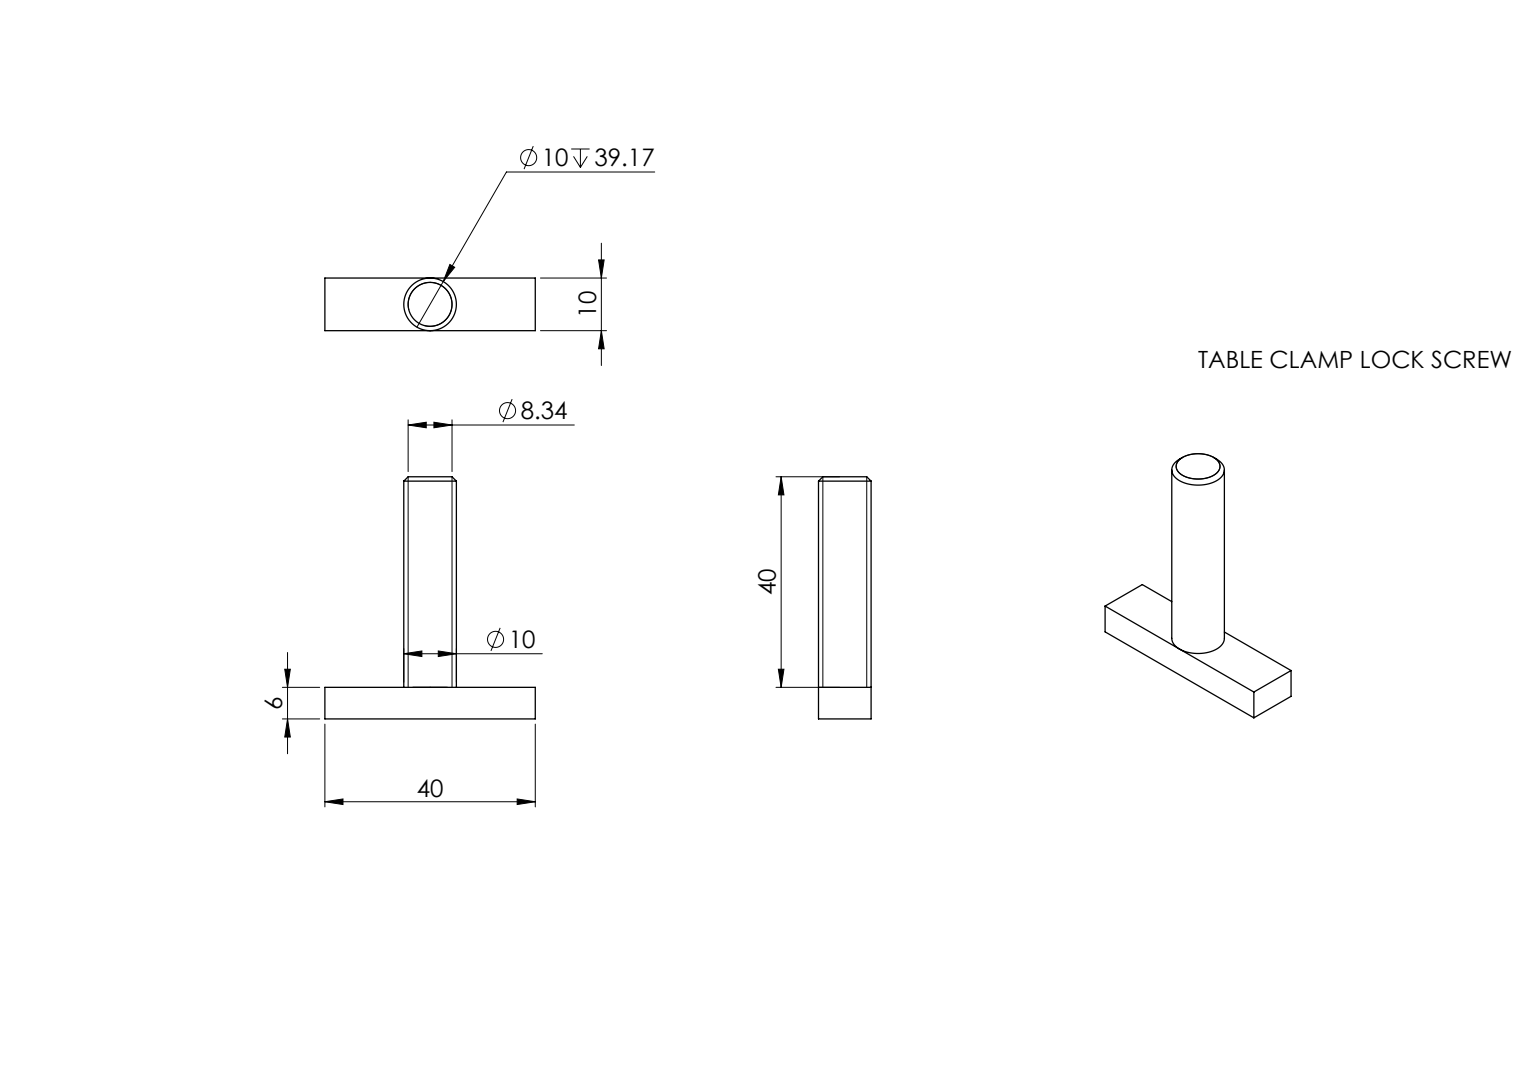
ISO-10303-21;
HEADER;
FILE_DESCRIPTION (('STEP AP214'),
    '1' );
FILE_NAME ('Table Clamp Lock Screw.step',
    '2026-10-22T10:02:39',
    ( '' ),
    ( '' ),
    'SwSTEP 2.0',
    'SolidWorks 2026',
    '' );
FILE_SCHEMA (( 'AUTOMOTIVE_DESIGN' ));
ENDSEC;

DATA;
#63=ADVANCED_FACE ( 'NONE', ( #6296 ), #11663, .F. ) ;
#65=DIRECTION ( 'NONE',  ( -0.000000000000000000, -1.000000000000000000, -0.000000000000000000 ) ) ;
#81=COLOUR_RGB ( '',0.8941176470588234615, 0.8941176470588234615, 0.8941176470588234615 ) ;
#86=LINE ( 'NONE', #1108, #4140 ) ;
#156=DIRECTION ( 'NONE',  ( -0.000000000000000000, -1.000000000000000000, -0.000000000000000000 ) ) ;
#174=FACE_OUTER_BOUND ( 'NONE', #11292, .T. ) ;
#257=( NAMED_UNIT ( * ) SI_UNIT ( $, .STERADIAN. ) SOLID_ANGLE_UNIT ( ) );
#287=DIRECTION ( 'NONE',  ( 0.000000000000000000, 0.000000000000000000, -1.000000000000000000 ) ) ;
#300=CARTESIAN_POINT ( 'NONE',  ( -20.00000000000003197, -57.00000000000000000, 5.000000000000000000 ) ) ;
#357=FACE_OUTER_BOUND ( 'NONE', #4501, .T. ) ;
#394=UNCERTAINTY_MEASURE_WITH_UNIT (LENGTH_MEASURE( 1.000000000000000082E-05 ), #5013, 'distance_accuracy_value', 'NONE');
#416=CLOSED_SHELL ( 'NONE', ( #7269, #9582, #2198, #63, #11043, #9304, #2244, #10765, #4629, #4313, #3244, #8345 ) ) ;
#432=EDGE_CURVE ( 'NONE', #3322, #5122, #11360, .T. ) ;
#533=CARTESIAN_POINT ( 'NONE',  ( -20.00000000000003197, -63.00000000000000000, 5.000000000000000000 ) ) ;
#646=DIRECTION ( 'NONE',  ( 0.000000000000000000, 0.000000000000000000, 1.000000000000000000 ) ) ;
#657=CARTESIAN_POINT ( 'NONE',  ( 0.000000000000000000, -57.00000000000000000, 0.000000000000000000 ) ) ;
#733=EDGE_CURVE ( 'NONE', #9917, #5658, #853, .T. ) ;
#777=DIRECTION ( 'NONE',  ( -0.000000000000000000, -1.000000000000000000, -0.000000000000000000 ) ) ;
#844=( GEOMETRIC_REPRESENTATION_CONTEXT ( 3 ) GLOBAL_UNCERTAINTY_ASSIGNED_CONTEXT ( ( #5921 ) ) GLOBAL_UNIT_ASSIGNED_CONTEXT ( ( #5850, #10497, #257 ) ) REPRESENTATION_CONTEXT ( 'NONE', 'WORKASPACE' ) );
#853=CIRCLE ( 'NONE', #2783, 4.171999999999999709 ) ;
#865=FACE_OUTER_BOUND ( 'NONE', #7245, .T. ) ;
#905=LINE ( 'NONE', #4465, #8956 ) ;
#995=ORIENTED_EDGE ( 'NONE', *, *, #8595, .F. ) ;
#1001=CARTESIAN_POINT ( 'NONE',  ( 0.000000000000000000, -17.82799999999998875, 0.000000000000000000 ) ) ;
#1089=CARTESIAN_POINT ( 'NONE',  ( 0.000000000000000000, -17.82799999999998875, -4.999999999999995559 ) ) ;
#1094=ORIENTED_EDGE ( 'NONE', *, *, #432, .T. ) ;
#1108=CARTESIAN_POINT ( 'NONE',  ( -20.00000000000003197, -57.00000000000000000, 5.000000000000000000 ) ) ;
#1155=AXIS2_PLACEMENT_3D ( 'NONE', #5306, #2664, #4410 ) ;
#1159=VECTOR ( 'NONE', #10817, 1000.000000000000000 ) ;
#1182=EDGE_CURVE ( 'NONE', #3322, #7121, #8405, .T. ) ;
#1184=( NAMED_UNIT ( * ) SI_UNIT ( $, .STERADIAN. ) SOLID_ANGLE_UNIT ( ) );
#1255=FACE_OUTER_BOUND ( 'NONE', #2174, .T. ) ;
#1282=LINE ( 'NONE', #10265, #7592 ) ;
#1303=ORIENTED_EDGE ( 'NONE', *, *, #1182, .F. ) ;
#1305=CARTESIAN_POINT ( 'NONE',  ( 19.99999999999996803, -63.00000000000000000, 5.000000000000000000 ) ) ;
#1346=CARTESIAN_POINT ( 'NONE',  ( 0.000000000000000000, -17.82799999999998875, -4.999999999999995559 ) ) ;
#1347=SURFACE_STYLE_USAGE ( .BOTH. , #2122 ) ;
#1383=DIRECTION ( 'NONE',  ( 1.000000000000000000, 0.000000000000000000, 0.000000000000000000 ) ) ;
#1405=FILL_AREA_STYLE ('',( #5909 ) ) ;
#1440=STYLED_ITEM ( 'NONE', ( #5732 ), #4566 ) ;
#1453=PRODUCT ( 'Table Clamp Lock Screw', 'Table Clamp Lock Screw', '', ( #9179 ) ) ;
#1565=ORIENTED_EDGE ( 'NONE', *, *, #10552, .T. ) ;
#1669=ORIENTED_EDGE ( 'NONE', *, *, #5875, .F. ) ;
#1676=CYLINDRICAL_SURFACE ( 'NONE', #10532, 4.999999999999997335 ) ;
#1688=ORIENTED_EDGE ( 'NONE', *, *, #5113, .T. ) ;
#1701=CARTESIAN_POINT ( 'NONE',  ( -20.00000000000003197, -63.00000000000000000, 5.000000000000000000 ) ) ;
#1708=CARTESIAN_POINT ( 'NONE',  ( 0.000000000000000000, -17.82799999999998875, 0.000000000000000000 ) ) ;
#1723=DIRECTION ( 'NONE',  ( -0.000000000000000000, -0.000000000000000000, -1.000000000000000000 ) ) ;
#1787=PLANE ( 'NONE',  #11606 ) ;
#1877=MECHANICAL_DESIGN_GEOMETRIC_PRESENTATION_REPRESENTATION('',(#6123),#11251);
#1892=ORIENTED_EDGE ( 'NONE', *, *, #4690, .T. ) ;
#1924=CARTESIAN_POINT ( 'NONE',  ( 6.123233995736761352E-16, -17.82799999999998875, 4.999999999999995559 ) ) ;
#2039=VECTOR ( 'NONE', #4198, 1000.000000000000000 ) ;
#2087=CARTESIAN_POINT ( 'NONE',  ( 0.000000000000000000, -17.82799999999998875, 0.000000000000000000 ) ) ;
#2122=SURFACE_SIDE_STYLE ('',( #9552 ) ) ;
#2174=EDGE_LOOP ( 'NONE', ( #11721, #10327, #3071, #9481 ) ) ;
#2197=PRODUCT_DEFINITION ( 'UNKNOWN', '', #10978, #3306 ) ;
#2198=ADVANCED_FACE ( 'NONE', ( #9905 ), #2546, .F. ) ;
#2216=EDGE_CURVE ( 'NONE', #2768, #9929, #10794, .T. ) ;
#2225=CIRCLE ( 'NONE', #4337, 4.171999999999999709 ) ;
#2244=ADVANCED_FACE ( 'NONE', ( #2605 ), #2729, .F. ) ;
#2410=ORIENTED_EDGE ( 'NONE', *, *, #8591, .F. ) ;
#2460=DIRECTION ( 'NONE',  ( -0.000000000000000000, -1.000000000000000000, -0.000000000000000000 ) ) ;
#2467=VECTOR ( 'NONE', #4475, 1000.000000000000000 ) ;
#2546=PLANE ( 'NONE',  #1155 ) ;
#2603=VERTEX_POINT ( 'NONE', #8563 ) ;
#2605=FACE_OUTER_BOUND ( 'NONE', #8879, .T. ) ;
#2664=DIRECTION ( 'NONE',  ( 0.000000000000000000, -1.000000000000000000, 0.000000000000000000 ) ) ;
#2671=EDGE_LOOP ( 'NONE', ( #8662, #1669, #10822, #1688 ) ) ;
#2696=ORIENTED_EDGE ( 'NONE', *, *, #11695, .T. ) ;
#2705=AXIS2_PLACEMENT_3D ( 'NONE', #6076, #10774, #8759 ) ;
#2729=PLANE ( 'NONE',  #7869 ) ;
#2768=VERTEX_POINT ( 'NONE', #1305 ) ;
#2783=AXIS2_PLACEMENT_3D ( 'NONE', #5496, #9145, #3695 ) ;
#2840=ORIENTED_EDGE ( 'NONE', *, *, #5067, .T. ) ;
#2859=CARTESIAN_POINT ( 'NONE',  ( 6.123233995736761352E-16, -17.82799999999998875, 4.999999999999995559 ) ) ;
#2946=EDGE_CURVE ( 'NONE', #9538, #5122, #7903, .T. ) ;
#2953=VECTOR ( 'NONE', #10579, 1000.000000000000000 ) ;
#3042=DIRECTION ( 'NONE',  ( -0.000000000000000000, -0.000000000000000000, -1.000000000000000000 ) ) ;
#3062=EDGE_CURVE ( 'NONE', #5122, #6726, #11232, .T. ) ;
#3071=ORIENTED_EDGE ( 'NONE', *, *, #9421, .F. ) ;
#3083=EDGE_CURVE ( 'NONE', #3150, #2603, #5811, .T. ) ;
#3089=( NAMED_UNIT ( * ) SI_UNIT ( $, .STERADIAN. ) SOLID_ANGLE_UNIT ( ) );
#3101=CARTESIAN_POINT ( 'NONE',  ( 19.99999999999996803, -57.00000000000000000, 5.000000000000000000 ) ) ;
#3108=( LENGTH_UNIT ( ) NAMED_UNIT ( * ) SI_UNIT ( .MILLI., .METRE. ) );
#3150=VERTEX_POINT ( 'NONE', #10342 ) ;
#3180=DIRECTION ( 'NONE',  ( -1.000000000000000000, 0.000000000000000000, -0.000000000000000000 ) ) ;
#3207=VERTEX_POINT ( 'NONE', #5199 ) ;
#3232=ORIENTED_EDGE ( 'NONE', *, *, #5875, .T. ) ;
#3244=ADVANCED_FACE ( 'NONE', ( #10687 ), #3557, .T. ) ;
#3264=VECTOR ( 'NONE', #3560, 1000.000000000000000 ) ;
#3306=PRODUCT_DEFINITION_CONTEXT ( 'detailed design', #10813, 'design' ) ;
#3322=VERTEX_POINT ( 'NONE', #1346 ) ;
#3442=CARTESIAN_POINT ( 'NONE',  ( 19.99999999999996803, -63.00000000000000000, 5.000000000000000000 ) ) ;
#3482=FACE_OUTER_BOUND ( 'NONE', #11135, .T. ) ;
#3511=LINE ( 'NONE', #7126, #2467 ) ;
#3544=( GEOMETRIC_REPRESENTATION_CONTEXT ( 3 ) GLOBAL_UNCERTAINTY_ASSIGNED_CONTEXT ( ( #394 ) ) GLOBAL_UNIT_ASSIGNED_CONTEXT ( ( #5013, #7644, #3089 ) ) REPRESENTATION_CONTEXT ( 'NONE', 'WORKASPACE' ) );
#3557=CONICAL_SURFACE ( 'NONE', #10242, 4.999999999999995559, 0.7853981633974530530 ) ;
#3560=DIRECTION ( 'NONE',  ( 0.000000000000000000, 1.000000000000000000, 0.000000000000000000 ) ) ;
#3591=EDGE_CURVE ( 'NONE', #9484, #9538, #1282, .T. ) ;
#3667=AXIS2_PLACEMENT_3D ( 'NONE', #5628, #156, #9508 ) ;
#3695=DIRECTION ( 'NONE',  ( 0.000000000000000000, 0.000000000000000000, -1.000000000000000000 ) ) ;
#3708=DIRECTION ( 'NONE',  ( 0.000000000000000000, -1.000000000000000000, 0.000000000000000000 ) ) ;
#3713=ORIENTED_EDGE ( 'NONE', *, *, #8804, .F. ) ;
#3749=DIRECTION ( 'NONE',  ( -1.000000000000000000, -0.000000000000000000, -0.000000000000000000 ) ) ;
#3761=CONICAL_SURFACE ( 'NONE', #5303, 4.999999999999995559, 0.7853981633974530530 ) ;
#3772=VECTOR ( 'NONE', #6533, 1000.000000000000000 ) ;
#3807=EDGE_CURVE ( 'NONE', #7121, #3322, #8159, .T. ) ;
#3818=ORIENTED_EDGE ( 'NONE', *, *, #3807, .T. ) ;
#3842=PLANE ( 'NONE',  #10150 ) ;
#3896=ORIENTED_EDGE ( 'NONE', *, *, #2216, .T. ) ;
#4021=CARTESIAN_POINT ( 'NONE',  ( 4.171999999999999709, -17.00000000000000000, 0.000000000000000000 ) ) ;
#4023=PLANE ( 'NONE',  #6481 ) ;
#4081=CARTESIAN_POINT ( 'NONE',  ( 0.000000000000000000, 0.000000000000000000, 5.000000000000000000 ) ) ;
#4122=CARTESIAN_POINT ( 'NONE',  ( 0.000000000000000000, -57.00000000000000000, -4.999999999999997335 ) ) ;
#4140=VECTOR ( 'NONE', #3749, 1000.000000000000000 ) ;
#4148=AXIS2_PLACEMENT_3D ( 'NONE', #7916, #5830, #6905 ) ;
#4172=SHAPE_REPRESENTATION ( 'Table Clamp Lock Screw', ( #4738 ), #844 ) ;
#4198=DIRECTION ( 'NONE',  ( -0.000000000000000000, -1.000000000000000000, -0.000000000000000000 ) ) ;
#4205=DIRECTION ( 'NONE',  ( 0.000000000000000000, 0.000000000000000000, -1.000000000000000000 ) ) ;
#4206=ORIENTED_EDGE ( 'NONE', *, *, #7278, .F. ) ;
#4265=DIRECTION ( 'NONE',  ( -0.000000000000000000, -1.000000000000000000, -0.000000000000000000 ) ) ;
#4281=DIRECTION ( 'NONE',  ( 0.000000000000000000, 0.000000000000000000, -1.000000000000000000 ) ) ;
#4295=CARTESIAN_POINT ( 'NONE',  ( 19.99999999999996803, -57.00000000000000000, 5.000000000000000000 ) ) ;
#4313=ADVANCED_FACE ( 'NONE', ( #174 ), #3842, .T. ) ;
#4337=AXIS2_PLACEMENT_3D ( 'NONE', #11160, #65, #8471 ) ;
#4357=ORIENTED_EDGE ( 'NONE', *, *, #3062, .T. ) ;
#4374=VECTOR ( 'NONE', #7623, 1000.000000000000000 ) ;
#4410=DIRECTION ( 'NONE',  ( 0.000000000000000000, -0.000000000000000000, -1.000000000000000000 ) ) ;
#4416=DIRECTION ( 'NONE',  ( -0.000000000000000000, -1.000000000000000000, -0.000000000000000000 ) ) ;
#4465=CARTESIAN_POINT ( 'NONE',  ( -20.00000000000003197, -63.00000000000000000, 5.000000000000000000 ) ) ;
#4475=DIRECTION ( 'NONE',  ( -0.000000000000000000, -0.000000000000000000, -1.000000000000000000 ) ) ;
#4501=EDGE_LOOP ( 'NONE', ( #3896, #5187, #1565, #9674, #2696 ) ) ;
#4518=ORIENTED_EDGE ( 'NONE', *, *, #8804, .T. ) ;
#4566=ADVANCED_BREP_SHAPE_REPRESENTATION ( '', ( #4740, #4738 ), #844 ) ;
#4603=DIRECTION ( 'NONE',  ( 0.000000000000000000, 0.000000000000000000, -1.000000000000000000 ) ) ;
#4629=ADVANCED_FACE ( 'NONE', ( #10941 ), #7142, .T. ) ;
#4636=ORIENTED_EDGE ( 'NONE', *, *, #9664, .F. ) ;
#4660=DIRECTION ( 'NONE',  ( 0.000000000000000000, 0.000000000000000000, -1.000000000000000000 ) ) ;
#4686=SHAPE_DEFINITION_REPRESENTATION ( #8071, #4172 ) ;
#4690=EDGE_CURVE ( 'NONE', #8651, #5122, #5392, .T. ) ;
#4724=CARTESIAN_POINT ( 'NONE',  ( 6.123233995736763324E-16, -57.00000000000000000, 4.999999999999997335 ) ) ;
#4738=AXIS2_PLACEMENT_3D ( 'NONE', #6164, #8011, #1383 ) ;
#4740=MANIFOLD_SOLID_BREP ( 'M10 Machine Threads Stud1', #416 ) ;
#4895=LINE ( 'NONE', #3101, #8810 ) ;
#5013=( LENGTH_UNIT ( ) NAMED_UNIT ( * ) SI_UNIT ( .MILLI., .METRE. ) );
#5020=AXIS2_PLACEMENT_3D ( 'NONE', #9927, #11725, #646 ) ;
#5067=EDGE_CURVE ( 'NONE', #2603, #9484, #11764, .T. ) ;
#5113=EDGE_CURVE ( 'NONE', #2768, #9484, #3511, .T. ) ;
#5122=VERTEX_POINT ( 'NONE', #9138 ) ;
#5187=ORIENTED_EDGE ( 'NONE', *, *, #8591, .T. ) ;
#5199=CARTESIAN_POINT ( 'NONE',  ( -20.00000000000003197, -57.00000000000000000, 5.000000000000000000 ) ) ;
#5236=CARTESIAN_POINT ( 'NONE',  ( -20.00000000000003197, -63.00000000000000000, -5.000000000000000000 ) ) ;
#5257=DIRECTION ( 'NONE',  ( 0.000000000000000000, 0.000000000000000000, -1.000000000000000000 ) ) ;
#5303=AXIS2_PLACEMENT_3D ( 'NONE', #1001, #10099, #4660 ) ;
#5306=CARTESIAN_POINT ( 'NONE',  ( -20.00000000000003197, -57.00000000000000000, 5.000000000000000000 ) ) ;
#5317=CARTESIAN_POINT ( 'NONE',  ( -20.00000000000003197, -63.00000000000000000, -5.000000000000000000 ) ) ;
#5362=CARTESIAN_POINT ( 'NONE',  ( 0.000000000000000000, -17.82799999999998875, 0.000000000000000000 ) ) ;
#5392=CIRCLE ( 'NONE', #3667, 5.000000000000000000 ) ;
#5398=CARTESIAN_POINT ( 'NONE',  ( -20.00000000000003197, -57.00000000000000000, 5.000000000000000000 ) ) ;
#5496=CARTESIAN_POINT ( 'NONE',  ( 0.000000000000000000, -17.00000000000000000, 0.000000000000000000 ) ) ;
#5502=LINE ( 'NONE', #2859, #1159 ) ;
#5533=AXIS2_PLACEMENT_3D ( 'NONE', #2087, #8507, #287 ) ;
#5567=FACE_OUTER_BOUND ( 'NONE', #9764, .T. ) ;
#5628=CARTESIAN_POINT ( 'NONE',  ( 0.000000000000000000, -57.00000000000000000, 0.000000000000000000 ) ) ;
#5629=CARTESIAN_POINT ( 'NONE',  ( 19.99999999999996803, -57.00000000000000000, -5.000000000000000000 ) ) ;
#5633=UNCERTAINTY_MEASURE_WITH_UNIT (LENGTH_MEASURE( 1.000000000000000082E-05 ), #3108, 'distance_accuracy_value', 'NONE');
#5658=VERTEX_POINT ( 'NONE', #11600 ) ;
#5663=ORIENTED_EDGE ( 'NONE', *, *, #10552, .F. ) ;
#5691=LINE ( 'NONE', #4724, #3772 ) ;
#5732=PRESENTATION_STYLE_ASSIGNMENT (( #1347 ) ) ;
#5811=LINE ( 'NONE', #8619, #10807 ) ;
#5830=DIRECTION ( 'NONE',  ( 1.000000000000000000, 0.000000000000000000, 0.000000000000000000 ) ) ;
#5850=( LENGTH_UNIT ( ) NAMED_UNIT ( * ) SI_UNIT ( .MILLI., .METRE. ) );
#5875=EDGE_CURVE ( 'NONE', #9929, #9538, #4895, .T. ) ;
#5909=FILL_AREA_STYLE_COLOUR ( '', #81 ) ;
#5921=UNCERTAINTY_MEASURE_WITH_UNIT (LENGTH_MEASURE( 1.000000000000000082E-05 ), #5850, 'distance_accuracy_value', 'NONE');
#5926=CARTESIAN_POINT ( 'NONE',  ( -20.00000000000003197, -57.00000000000000000, -5.000000000000000000 ) ) ;
#5934=DIRECTION ( 'NONE',  ( -1.000000000000000000, -0.000000000000000000, -0.000000000000000000 ) ) ;
#6076=CARTESIAN_POINT ( 'NONE',  ( 0.000000000000000000, -57.00000000000000000, 0.000000000000000000 ) ) ;
#6084=ORIENTED_EDGE ( 'NONE', *, *, #11695, .F. ) ;
#6098=DIRECTION ( 'NONE',  ( -0.000000000000000000, -0.000000000000000000, -1.000000000000000000 ) ) ;
#6108=ORIENTED_EDGE ( 'NONE', *, *, #1182, .T. ) ;
#6123=STYLED_ITEM('',(#11895),#4740);
#6127=DIRECTION ( 'NONE',  ( 0.000000000000000000, 0.000000000000000000, -1.000000000000000000 ) ) ;
#6133=ORIENTED_EDGE ( 'NONE', *, *, #9063, .F. ) ;
#6164=CARTESIAN_POINT ( 'NONE',  ( 0.000000000000000000, 0.000000000000000000, 0.000000000000000000 ) ) ;
#6296=FACE_OUTER_BOUND ( 'NONE', #2671, .T. ) ;
#6358=AXIS2_PLACEMENT_3D ( 'NONE', #8874, #2460, #6127 ) ;
#6371=ORIENTED_EDGE ( 'NONE', *, *, #2946, .T. ) ;
#6386=DIRECTION ( 'NONE',  ( 0.000000000000000000, 1.000000000000000000, 0.000000000000000000 ) ) ;
#6409=DIRECTION ( 'NONE',  ( -1.000000000000000000, 0.000000000000000000, -0.000000000000000000 ) ) ;
#6481=AXIS2_PLACEMENT_3D ( 'NONE', #4081, #11371, #3180 ) ;
#6532=VECTOR ( 'NONE', #1723, 1000.000000000000000 ) ;
#6533=DIRECTION ( 'NONE',  ( -0.000000000000000000, -1.000000000000000000, -0.000000000000000000 ) ) ;
#6544=ORIENTED_EDGE ( 'NONE', *, *, #432, .F. ) ;
#6570=ORIENTED_EDGE ( 'NONE', *, *, #3591, .F. ) ;
#6626=DIRECTION ( 'NONE',  ( 0.000000000000000000, -0.000000000000000000, 1.000000000000000000 ) ) ;
#6726=VERTEX_POINT ( 'NONE', #11747 ) ;
#6732=DIRECTION ( 'NONE',  ( 0.000000000000000000, 1.000000000000000000, 0.000000000000000000 ) ) ;
#6763=ORIENTED_EDGE ( 'NONE', *, *, #3083, .T. ) ;
#6905=DIRECTION ( 'NONE',  ( 0.000000000000000000, 0.000000000000000000, -1.000000000000000000 ) ) ;
#7121=VERTEX_POINT ( 'NONE', #1924 ) ;
#7126=CARTESIAN_POINT ( 'NONE',  ( 19.99999999999996803, -63.00000000000000000, 5.000000000000000000 ) ) ;
#7129=ORIENTED_EDGE ( 'NONE', *, *, #733, .F. ) ;
#7142=PLANE ( 'NONE',  #8258 ) ;
#7205=DIRECTION ( 'NONE',  ( 0.000000000000000000, -0.000000000000000000, -1.000000000000000000 ) ) ;
#7245=EDGE_LOOP ( 'NONE', ( #4636, #3818, #1094, #10976 ) ) ;
#7269=ADVANCED_FACE ( 'NONE', ( #7864 ), #1676, .T. ) ;
#7278=EDGE_CURVE ( 'NONE', #5122, #8651, #11677, .T. ) ;
#7462=ORIENTED_EDGE ( 'NONE', *, *, #733, .T. ) ;
#7592=VECTOR ( 'NONE', #9430, 1000.000000000000000 ) ;
#7603=( NAMED_UNIT ( * ) PLANE_ANGLE_UNIT ( ) SI_UNIT ( $, .RADIAN. ) );
#7623=DIRECTION ( 'NONE',  ( -1.000000000000000000, -0.000000000000000000, -0.000000000000000000 ) ) ;
#7644=( NAMED_UNIT ( * ) PLANE_ANGLE_UNIT ( ) SI_UNIT ( $, .RADIAN. ) );
#7659=EDGE_CURVE ( 'NONE', #9917, #7121, #5502, .T. ) ;
#7688=EDGE_CURVE ( 'NONE', #3207, #6726, #9925, .T. ) ;
#7776=VECTOR ( 'NONE', #5934, 1000.000000000000000 ) ;
#7864=FACE_OUTER_BOUND ( 'NONE', #8727, .T. ) ;
#7869=AXIS2_PLACEMENT_3D ( 'NONE', #1701, #6386, #6626 ) ;
#7903=LINE ( 'NONE', #11593, #7776 ) ;
#7916=CARTESIAN_POINT ( 'NONE',  ( -20.00000000000003197, -63.00000000000000000, 5.000000000000000000 ) ) ;
#8011=DIRECTION ( 'NONE',  ( 0.000000000000000000, 0.000000000000000000, 1.000000000000000000 ) ) ;
#8031=CARTESIAN_POINT ( 'NONE',  ( 19.99999999999996803, -63.00000000000000000, -5.000000000000000000 ) ) ;
#8058=ORIENTED_EDGE ( 'NONE', *, *, #5067, .F. ) ;
#8071=PRODUCT_DEFINITION_SHAPE ( 'NONE', 'NONE',  #2197 ) ;
#8126=ORIENTED_EDGE ( 'NONE', *, *, #3062, .F. ) ;
#8139=MECHANICAL_DESIGN_GEOMETRIC_PRESENTATION_REPRESENTATION('',(#1440),#3544);
#8159=CIRCLE ( 'NONE', #9684, 4.999999999999995559 ) ;
#8258=AXIS2_PLACEMENT_3D ( 'NONE', #11780, #4603, #6409 ) ;
#8298=EDGE_LOOP ( 'NONE', ( #10077, #7462, #4518, #11738 ) ) ;
#8345=ADVANCED_FACE ( 'NONE', ( #865 ), #9592, .T. ) ;
#8405=CIRCLE ( 'NONE', #5533, 4.999999999999995559 ) ;
#8406=DIRECTION ( 'NONE',  ( 0.000000000000000000, -0.7071067811865441310, -0.7071067811865507924 ) ) ;
#8471=DIRECTION ( 'NONE',  ( 0.000000000000000000, 0.000000000000000000, -1.000000000000000000 ) ) ;
#8481=SHAPE_REPRESENTATION_RELATIONSHIP ( 'NONE' , 'NONE' ,  #4172, #4566 ) ;
#8507=DIRECTION ( 'NONE',  ( -0.000000000000000000, -1.000000000000000000, -0.000000000000000000 ) ) ;
#8517=LINE ( 'NONE', #300, #4374 ) ;
#8563=CARTESIAN_POINT ( 'NONE',  ( -20.00000000000003197, -63.00000000000000000, -5.000000000000000000 ) ) ;
#8591=EDGE_CURVE ( 'NONE', #9929, #8651, #86, .T. ) ;
#8595=EDGE_CURVE ( 'NONE', #5658, #9917, #2225, .T. ) ;
#8619=CARTESIAN_POINT ( 'NONE',  ( -20.00000000000003197, -63.00000000000000000, 5.000000000000000000 ) ) ;
#8651=VERTEX_POINT ( 'NONE', #10375 ) ;
#8662=ORIENTED_EDGE ( 'NONE', *, *, #3591, .T. ) ;
#8725=VECTOR ( 'NONE', #9506, 1000.000000000000000 ) ;
#8727=EDGE_LOOP ( 'NONE', ( #6108, #10147, #4206, #6544 ) ) ;
#8751=LINE ( 'NONE', #533, #2039 ) ;
#8759=DIRECTION ( 'NONE',  ( 0.000000000000000000, 0.000000000000000000, -1.000000000000000000 ) ) ;
#8804=EDGE_CURVE ( 'NONE', #5658, #3322, #9296, .T. ) ;
#8810=VECTOR ( 'NONE', #6098, 1000.000000000000000 ) ;
#8874=CARTESIAN_POINT ( 'NONE',  ( 0.000000000000000000, -57.00000000000000000, 0.000000000000000000 ) ) ;
#8879=EDGE_LOOP ( 'NONE', ( #2840, #9618, #6084, #6763 ) ) ;
#8956=VECTOR ( 'NONE', #9844, 1000.000000000000000 ) ;
#8971=CARTESIAN_POINT ( 'NONE',  ( 5.616230220889759479E-16, -17.00000000000000000, 4.171999999999999709 ) ) ;
#9002=LINE ( 'NONE', #5236, #9700 ) ;
#9028=DIRECTION ( 'NONE',  ( 1.000000000000000000, 0.000000000000000000, 0.000000000000000000 ) ) ;
#9063=EDGE_CURVE ( 'NONE', #6726, #2603, #9002, .T. ) ;
#9091=CARTESIAN_POINT ( 'NONE',  ( -20.00000000000003197, -57.00000000000000000, 5.000000000000000000 ) ) ;
#9126=EDGE_LOOP ( 'NONE', ( #6570, #8058, #6133, #8126, #10673 ) ) ;
#9138=CARTESIAN_POINT ( 'NONE',  ( 0.000000000000000000, -57.00000000000000000, -5.000000000000000000 ) ) ;
#9145=DIRECTION ( 'NONE',  ( -0.000000000000000000, -1.000000000000000000, -0.000000000000000000 ) ) ;
#9179=PRODUCT_CONTEXT ( 'NONE', #10888, 'mechanical' ) ;
#9296=LINE ( 'NONE', #1089, #9689 ) ;
#9304=ADVANCED_FACE ( 'NONE', ( #1255 ), #11429, .F. ) ;
#9421=EDGE_CURVE ( 'NONE', #3207, #3150, #8751, .T. ) ;
#9430=DIRECTION ( 'NONE',  ( 0.000000000000000000, 1.000000000000000000, 0.000000000000000000 ) ) ;
#9481=ORIENTED_EDGE ( 'NONE', *, *, #7688, .T. ) ;
#9484=VERTEX_POINT ( 'NONE', #8031 ) ;
#9506=DIRECTION ( 'NONE',  ( -1.000000000000000000, -0.000000000000000000, -0.000000000000000000 ) ) ;
#9508=DIRECTION ( 'NONE',  ( 0.000000000000000000, 0.000000000000000000, -1.000000000000000000 ) ) ;
#9533=ORIENTED_EDGE ( 'NONE', *, *, #7659, .T. ) ;
#9538=VERTEX_POINT ( 'NONE', #5629 ) ;
#9552=SURFACE_STYLE_FILL_AREA ( #1405 ) ;
#9559=EDGE_LOOP ( 'NONE', ( #6371, #11255, #2410, #3232 ) ) ;
#9582=ADVANCED_FACE ( 'NONE', ( #5567 ), #3761, .T. ) ;
#9592=CYLINDRICAL_SURFACE ( 'NONE', #6358, 4.999999999999997335 ) ;
#9618=ORIENTED_EDGE ( 'NONE', *, *, #5113, .F. ) ;
#9664=EDGE_CURVE ( 'NONE', #7121, #8651, #5691, .T. ) ;
#9674=ORIENTED_EDGE ( 'NONE', *, *, #9421, .T. ) ;
#9684=AXIS2_PLACEMENT_3D ( 'NONE', #5362, #9723, #4281 ) ;
#9689=VECTOR ( 'NONE', #8406, 1000.000000000000000 ) ;
#9700=VECTOR ( 'NONE', #777, 1000.000000000000000 ) ;
#9723=DIRECTION ( 'NONE',  ( -0.000000000000000000, -1.000000000000000000, -0.000000000000000000 ) ) ;
#9764=EDGE_LOOP ( 'NONE', ( #11322, #9533, #1303, #3713 ) ) ;
#9844=DIRECTION ( 'NONE',  ( 1.000000000000000000, 0.000000000000000000, 0.000000000000000000 ) ) ;
#9905=FACE_OUTER_BOUND ( 'NONE', #9559, .T. ) ;
#9917=VERTEX_POINT ( 'NONE', #8971 ) ;
#9925=LINE ( 'NONE', #9091, #6532 ) ;
#9927=CARTESIAN_POINT ( 'NONE',  ( 19.99999999999996803, -63.00000000000000000, 5.000000000000000000 ) ) ;
#9929=VERTEX_POINT ( 'NONE', #4295 ) ;
#10077=ORIENTED_EDGE ( 'NONE', *, *, #7659, .F. ) ;
#10099=DIRECTION ( 'NONE',  ( -0.000000000000000000, -1.000000000000000000, -0.000000000000000000 ) ) ;
#10147=ORIENTED_EDGE ( 'NONE', *, *, #9664, .T. ) ;
#10150=AXIS2_PLACEMENT_3D ( 'NONE', #4021, #6732, #11188 ) ;
#10242=AXIS2_PLACEMENT_3D ( 'NONE', #1708, #4416, #5257 ) ;
#10265=CARTESIAN_POINT ( 'NONE',  ( 19.99999999999996803, -63.00000000000000000, -5.000000000000000000 ) ) ;
#10327=ORIENTED_EDGE ( 'NONE', *, *, #3083, .F. ) ;
#10342=CARTESIAN_POINT ( 'NONE',  ( -20.00000000000003197, -63.00000000000000000, 5.000000000000000000 ) ) ;
#10375=CARTESIAN_POINT ( 'NONE',  ( 0.000000000000000000, -57.00000000000000000, 5.000000000000000000 ) ) ;
#10497=( NAMED_UNIT ( * ) PLANE_ANGLE_UNIT ( ) SI_UNIT ( $, .RADIAN. ) );
#10532=AXIS2_PLACEMENT_3D ( 'NONE', #657, #4265, #4205 ) ;
#10552=EDGE_CURVE ( 'NONE', #8651, #3207, #8517, .T. ) ;
#10579=DIRECTION ( 'NONE',  ( -0.000000000000000000, -1.000000000000000000, -0.000000000000000000 ) ) ;
#10673=ORIENTED_EDGE ( 'NONE', *, *, #2946, .F. ) ;
#10675=VECTOR ( 'NONE', #9028, 1000.000000000000000 ) ;
#10687=FACE_OUTER_BOUND ( 'NONE', #8298, .T. ) ;
#10765=ADVANCED_FACE ( 'NONE', ( #357 ), #4023, .F. ) ;
#10774=DIRECTION ( 'NONE',  ( -0.000000000000000000, -1.000000000000000000, -0.000000000000000000 ) ) ;
#10794=LINE ( 'NONE', #3442, #3264 ) ;
#10807=VECTOR ( 'NONE', #3042, 1000.000000000000000 ) ;
#10813=APPLICATION_CONTEXT ( 'automotive_design' ) ;
#10817=DIRECTION ( 'NONE',  ( 8.659560562354974766E-17, -0.7071067811865441310, 0.7071067811865507924 ) ) ;
#10822=ORIENTED_EDGE ( 'NONE', *, *, #2216, .F. ) ;
#10888=APPLICATION_CONTEXT ( 'automotive_design' ) ;
#10941=FACE_OUTER_BOUND ( 'NONE', #9126, .T. ) ;
#10976=ORIENTED_EDGE ( 'NONE', *, *, #4690, .F. ) ;
#10978=PRODUCT_DEFINITION_FORMATION_WITH_SPECIFIED_SOURCE ( 'ANY', '', #1453, .NOT_KNOWN. ) ;
#11043=ADVANCED_FACE ( 'NONE', ( #3482 ), #1787, .F. ) ;
#11135=EDGE_LOOP ( 'NONE', ( #5663, #1892, #4357, #11152 ) ) ;
#11152=ORIENTED_EDGE ( 'NONE', *, *, #7688, .F. ) ;
#11160=CARTESIAN_POINT ( 'NONE',  ( 0.000000000000000000, -17.00000000000000000, 0.000000000000000000 ) ) ;
#11188=DIRECTION ( 'NONE',  ( 0.000000000000000000, -0.000000000000000000, 1.000000000000000000 ) ) ;
#11232=LINE ( 'NONE', #5926, #8725 ) ;
#11251=( GEOMETRIC_REPRESENTATION_CONTEXT ( 3 ) GLOBAL_UNCERTAINTY_ASSIGNED_CONTEXT ( ( #5633 ) ) GLOBAL_UNIT_ASSIGNED_CONTEXT ( ( #3108, #7603, #1184 ) ) REPRESENTATION_CONTEXT ( 'NONE', 'WORKASPACE' ) );
#11255=ORIENTED_EDGE ( 'NONE', *, *, #7278, .T. ) ;
#11292=EDGE_LOOP ( 'NONE', ( #995, #7129 ) ) ;
#11322=ORIENTED_EDGE ( 'NONE', *, *, #8595, .T. ) ;
#11360=LINE ( 'NONE', #4122, #2953 ) ;
#11371=DIRECTION ( 'NONE',  ( 0.000000000000000000, 0.000000000000000000, -1.000000000000000000 ) ) ;
#11429=PLANE ( 'NONE',  #4148 ) ;
#11593=CARTESIAN_POINT ( 'NONE',  ( -20.00000000000003197, -57.00000000000000000, -5.000000000000000000 ) ) ;
#11600=CARTESIAN_POINT ( 'NONE',  ( 0.000000000000000000, -17.00000000000000000, -4.171999999999999709 ) ) ;
#11606=AXIS2_PLACEMENT_3D ( 'NONE', #5398, #3708, #7205 ) ;
#11663=PLANE ( 'NONE',  #5020 ) ;
#11677=CIRCLE ( 'NONE', #2705, 5.000000000000000000 ) ;
#11695=EDGE_CURVE ( 'NONE', #3150, #2768, #905, .T. ) ;
#11721=ORIENTED_EDGE ( 'NONE', *, *, #9063, .T. ) ;
#11725=DIRECTION ( 'NONE',  ( -1.000000000000000000, 0.000000000000000000, 0.000000000000000000 ) ) ;
#11738=ORIENTED_EDGE ( 'NONE', *, *, #3807, .F. ) ;
#11747=CARTESIAN_POINT ( 'NONE',  ( -20.00000000000003197, -57.00000000000000000, -5.000000000000000000 ) ) ;
#11764=LINE ( 'NONE', #5317, #10675 ) ;
#11780=CARTESIAN_POINT ( 'NONE',  ( 0.000000000000000000, 0.000000000000000000, -5.000000000000000000 ) ) ;
#11889=COLOUR_RGB('Black',0.12,0.14,0.17);
#11890=FILL_AREA_STYLE_COLOUR('',#11889);
#11891=FILL_AREA_STYLE('',(#11890));
#11892=SURFACE_STYLE_FILL_AREA(#11891);
#11893=SURFACE_SIDE_STYLE('',(#11892));
#11894=SURFACE_STYLE_USAGE(.BOTH.,#11893);
#11895=PRESENTATION_STYLE_ASSIGNMENT((#11894));
ENDSEC;
END-ISO-10303-21;
